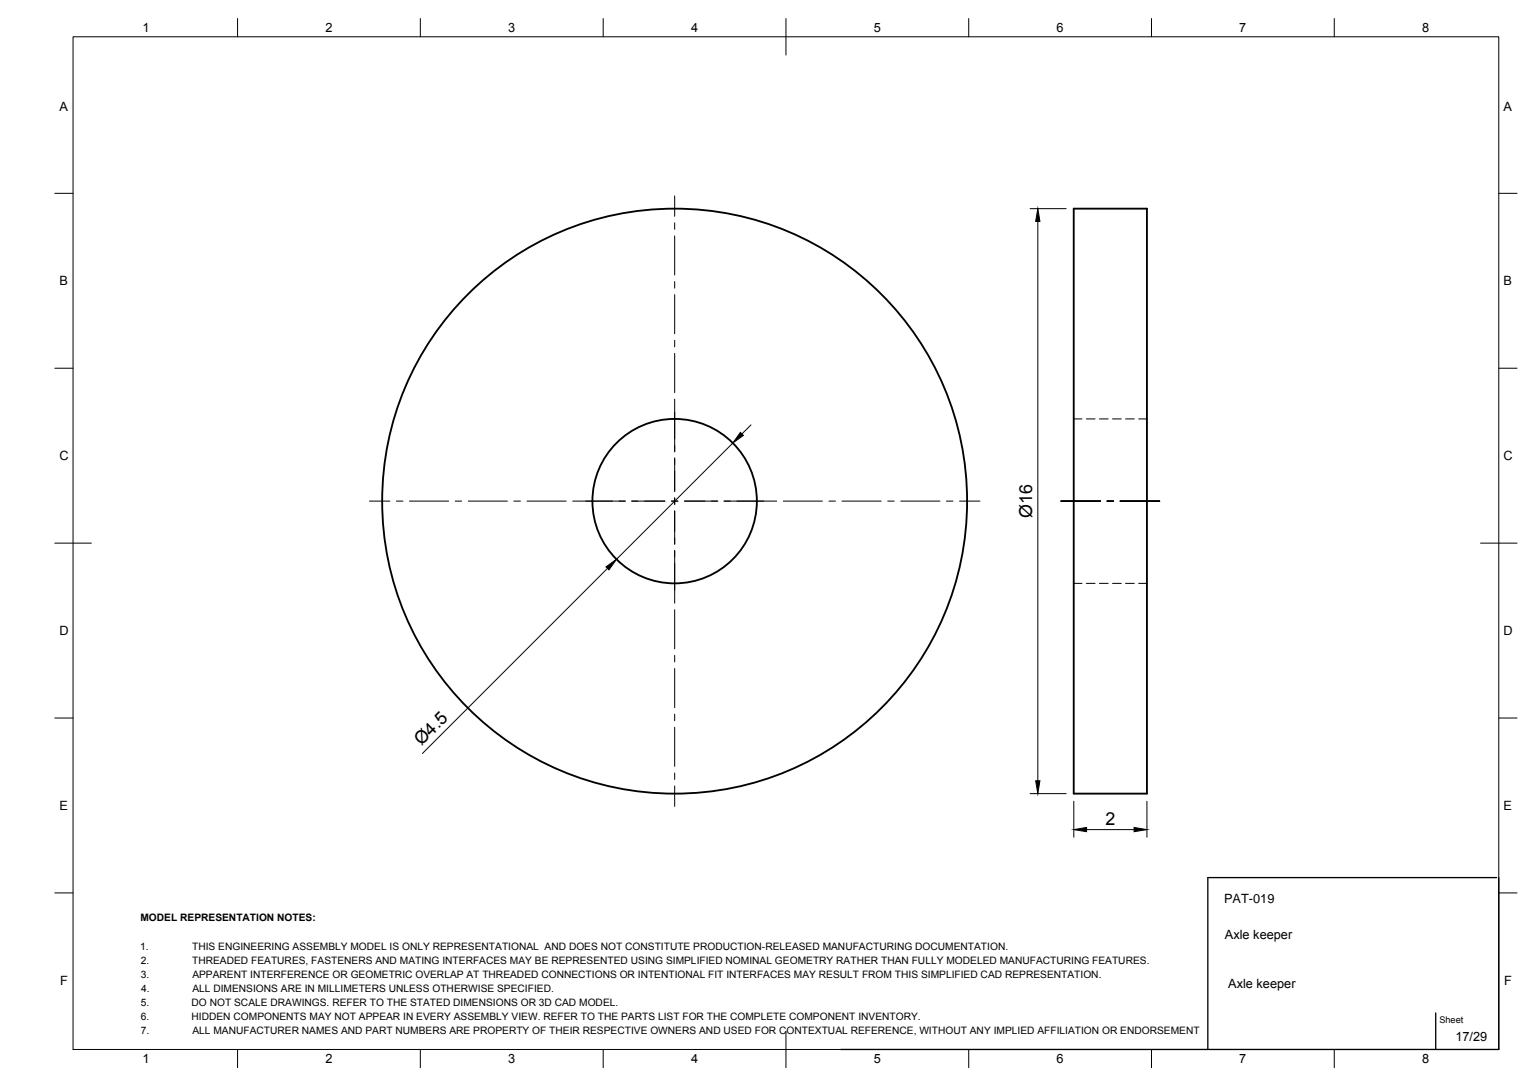
ISO-10303-21;
HEADER;
/* Generated by software containing ST-Developer
 * from STEP Tools, Inc. (www.steptools.com) 
 */

FILE_DESCRIPTION(
/* description */ ('Caster wheel assembly'),
/* implementation_level */ '2;1');

FILE_NAME(
/* name */ 'Axle keeper.step',
/* time_stamp */ '2026-10-28T03:23:56-07:00',
/* author */ (''),
/* organization */ (''),
/* preprocessor_version */ 'ST-DEVELOPER v20.2',
/* originating_system */ 'Autodesk Translation Framework v15.17.0.0',
/* authorisation */ '');

FILE_SCHEMA (('AUTOMOTIVE_DESIGN { 1 0 10303 214 3 1 1 }'));
ENDSEC;

DATA;
#10=MECHANICAL_DESIGN_GEOMETRIC_PRESENTATION_REPRESENTATION('',(#234),#5385);
#190=SHAPE_REPRESENTATION_RELATIONSHIP('SRR','None',#5486,#212);
#212=ADVANCED_BREP_SHAPE_REPRESENTATION('',(#264),#5373);
#234=STYLED_ITEM('',(#5672),#264);
#264=MANIFOLD_SOLID_BREP('Body1',#2661);
#313=FACE_BOUND('',#705,.T.);
#314=FACE_BOUND('',#707,.T.);
#383=PLANE('',#3091);
#384=PLANE('',#3092);
#502=FACE_OUTER_BOUND('',#702,.T.);
#503=FACE_OUTER_BOUND('',#703,.T.);
#504=FACE_OUTER_BOUND('',#704,.T.);
#505=FACE_OUTER_BOUND('',#706,.T.);
#702=EDGE_LOOP('',(#2096,#2097,#2098,#2099));
#703=EDGE_LOOP('',(#2100,#2101,#2102,#2103));
#704=EDGE_LOOP('',(#2104));
#705=EDGE_LOOP('',(#2105));
#706=EDGE_LOOP('',(#2106));
#707=EDGE_LOOP('',(#2107));
#894=LINE('',#4591,#1028);
#895=LINE('',#4597,#1029);
#1028=VECTOR('',#3717,0.225);
#1029=VECTOR('',#3724,0.8);
#1137=CIRCLE('',#3086,0.225);
#1138=CIRCLE('',#3087,0.225);
#1139=CIRCLE('',#3089,0.8);
#1140=CIRCLE('',#3090,0.8);
#1340=VERTEX_POINT('',#4588);
#1341=VERTEX_POINT('',#4590);
#1342=VERTEX_POINT('',#4594);
#1343=VERTEX_POINT('',#4596);
#1616=EDGE_CURVE('',#1340,#1340,#1137,.T.);
#1617=EDGE_CURVE('',#1340,#1341,#894,.T.);
#1618=EDGE_CURVE('',#1341,#1341,#1138,.T.);
#1619=EDGE_CURVE('',#1342,#1342,#1139,.T.);
#1620=EDGE_CURVE('',#1342,#1343,#895,.T.);
#1621=EDGE_CURVE('',#1343,#1343,#1140,.T.);
#2096=ORIENTED_EDGE('',*,*,#1616,.F.);
#2097=ORIENTED_EDGE('',*,*,#1617,.T.);
#2098=ORIENTED_EDGE('',*,*,#1618,.T.);
#2099=ORIENTED_EDGE('',*,*,#1617,.F.);
#2100=ORIENTED_EDGE('',*,*,#1619,.F.);
#2101=ORIENTED_EDGE('',*,*,#1620,.T.);
#2102=ORIENTED_EDGE('',*,*,#1621,.T.);
#2103=ORIENTED_EDGE('',*,*,#1620,.F.);
#2104=ORIENTED_EDGE('',*,*,#1619,.T.);
#2105=ORIENTED_EDGE('',*,*,#1616,.T.);
#2106=ORIENTED_EDGE('',*,*,#1621,.F.);
#2107=ORIENTED_EDGE('',*,*,#1618,.F.);
#2457=CYLINDRICAL_SURFACE('',#3085,0.225);
#2458=CYLINDRICAL_SURFACE('',#3088,0.8);
#2562=ADVANCED_FACE('',(#502),#2457,.F.);
#2563=ADVANCED_FACE('',(#503),#2458,.T.);
#2564=ADVANCED_FACE('',(#504,#313),#383,.T.);
#2565=ADVANCED_FACE('',(#505,#314),#384,.F.);
#2661=CLOSED_SHELL('',(#2562,#2563,#2564,#2565));
#3084=AXIS2_PLACEMENT_3D('',#4586,#3711,#3712);
#3085=AXIS2_PLACEMENT_3D('',#4587,#3713,#3714);
#3086=AXIS2_PLACEMENT_3D('',#4589,#3715,#3716);
#3087=AXIS2_PLACEMENT_3D('',#4592,#3718,#3719);
#3088=AXIS2_PLACEMENT_3D('',#4593,#3720,#3721);
#3089=AXIS2_PLACEMENT_3D('',#4595,#3722,#3723);
#3090=AXIS2_PLACEMENT_3D('',#4598,#3725,#3726);
#3091=AXIS2_PLACEMENT_3D('',#4599,#3727,#3728);
#3092=AXIS2_PLACEMENT_3D('',#4600,#3729,#3730);
#3711=DIRECTION('axis',(0.,0.,1.));
#3712=DIRECTION('refdir',(1.,0.,0.));
#3713=DIRECTION('center_axis',(0.,1.,0.));
#3714=DIRECTION('ref_axis',(1.,0.,0.));
#3715=DIRECTION('center_axis',(0.,-1.,0.));
#3716=DIRECTION('ref_axis',(1.,0.,0.));
#3717=DIRECTION('',(0.,-1.,0.));
#3718=DIRECTION('center_axis',(0.,-1.,0.));
#3719=DIRECTION('ref_axis',(1.,0.,0.));
#3720=DIRECTION('center_axis',(0.,1.,0.));
#3721=DIRECTION('ref_axis',(1.,0.,0.));
#3722=DIRECTION('center_axis',(0.,1.,0.));
#3723=DIRECTION('ref_axis',(1.,0.,0.));
#3724=DIRECTION('',(0.,-1.,0.));
#3725=DIRECTION('center_axis',(0.,1.,0.));
#3726=DIRECTION('ref_axis',(1.,0.,0.));
#3727=DIRECTION('center_axis',(0.,1.,0.));
#3728=DIRECTION('ref_axis',(1.,0.,0.));
#3729=DIRECTION('center_axis',(0.,1.,0.));
#3730=DIRECTION('ref_axis',(1.,0.,0.));
#4586=CARTESIAN_POINT('',(0.,0.,0.));
#4587=CARTESIAN_POINT('Origin',(0.,2.2,4.));
#4588=CARTESIAN_POINT('',(-0.225,2.4,4.));
#4589=CARTESIAN_POINT('Origin',(0.,2.4,4.));
#4590=CARTESIAN_POINT('',(-0.225,2.2,4.));
#4591=CARTESIAN_POINT('',(-0.225,2.2,4.));
#4592=CARTESIAN_POINT('Origin',(0.,2.2,4.));
#4593=CARTESIAN_POINT('Origin',(0.,2.2,4.));
#4594=CARTESIAN_POINT('',(-0.8,2.4,4.));
#4595=CARTESIAN_POINT('Origin',(0.,2.4,4.));
#4596=CARTESIAN_POINT('',(-0.8,2.2,4.));
#4597=CARTESIAN_POINT('',(-0.8,2.2,4.));
#4598=CARTESIAN_POINT('Origin',(0.,2.2,4.));
#4599=CARTESIAN_POINT('Origin',(0.,2.4,4.));
#4600=CARTESIAN_POINT('Origin',(0.,2.2,4.));
#5345=UNCERTAINTY_MEASURE_WITH_UNIT(LENGTH_MEASURE(0.001),#5386,
'DISTANCE_ACCURACY_VALUE',
'Maximum model space distance between geometric entities at asserted c
onnectivities');
#5357=UNCERTAINTY_MEASURE_WITH_UNIT(LENGTH_MEASURE(0.001),#5386,
'DISTANCE_ACCURACY_VALUE',
'Maximum model space distance between geometric entities at asserted c
onnectivities');
#5373=(
GEOMETRIC_REPRESENTATION_CONTEXT(3)
GLOBAL_UNCERTAINTY_ASSIGNED_CONTEXT((#5345))
GLOBAL_UNIT_ASSIGNED_CONTEXT((#5386,#5388,#5389))
REPRESENTATION_CONTEXT('','3D')
);
#5385=(
GEOMETRIC_REPRESENTATION_CONTEXT(3)
GLOBAL_UNCERTAINTY_ASSIGNED_CONTEXT((#5357))
GLOBAL_UNIT_ASSIGNED_CONTEXT((#5386,#5388,#5389))
REPRESENTATION_CONTEXT('','3D')
);
#5386=(
LENGTH_UNIT()
NAMED_UNIT(*)
SI_UNIT(.CENTI.,.METRE.)
);
#5388=(
NAMED_UNIT(*)
PLANE_ANGLE_UNIT()
SI_UNIT($,.RADIAN.)
);
#5389=(
NAMED_UNIT(*)
SI_UNIT($,.STERADIAN.)
SOLID_ANGLE_UNIT()
);
#5405=SHAPE_DEFINITION_REPRESENTATION(#5437,#5486);
#5437=PRODUCT_DEFINITION_SHAPE('',$,#5514);
#5486=SHAPE_REPRESENTATION('',(#3084),#5373);
#5498=PRODUCT_DEFINITION_CONTEXT('part definition',#5581,'design');
#5514=PRODUCT_DEFINITION('Axle keeper','Axle keeper',#5541,#5498);
#5541=PRODUCT_DEFINITION_FORMATION('',$,#5598);
#5581=APPLICATION_CONTEXT(
'Core Data for Automotive Mechanical Design Process');
#5582=PRODUCT_CONTEXT('part definition',#5581,'mechanical');
#5598=PRODUCT('Axle keeper','Axle keeper','Axle keeper',(#5582));
#5666=COLOUR_RGB('Grey',0.48,0.52,0.57);
#5667=FILL_AREA_STYLE_COLOUR('',#5666);
#5668=FILL_AREA_STYLE('',(#5667));
#5669=SURFACE_STYLE_FILL_AREA(#5668);
#5670=SURFACE_SIDE_STYLE('',(#5669));
#5671=SURFACE_STYLE_USAGE(.BOTH.,#5670);
#5672=PRESENTATION_STYLE_ASSIGNMENT((#5671));
ENDSEC;
END-ISO-10303-21;
